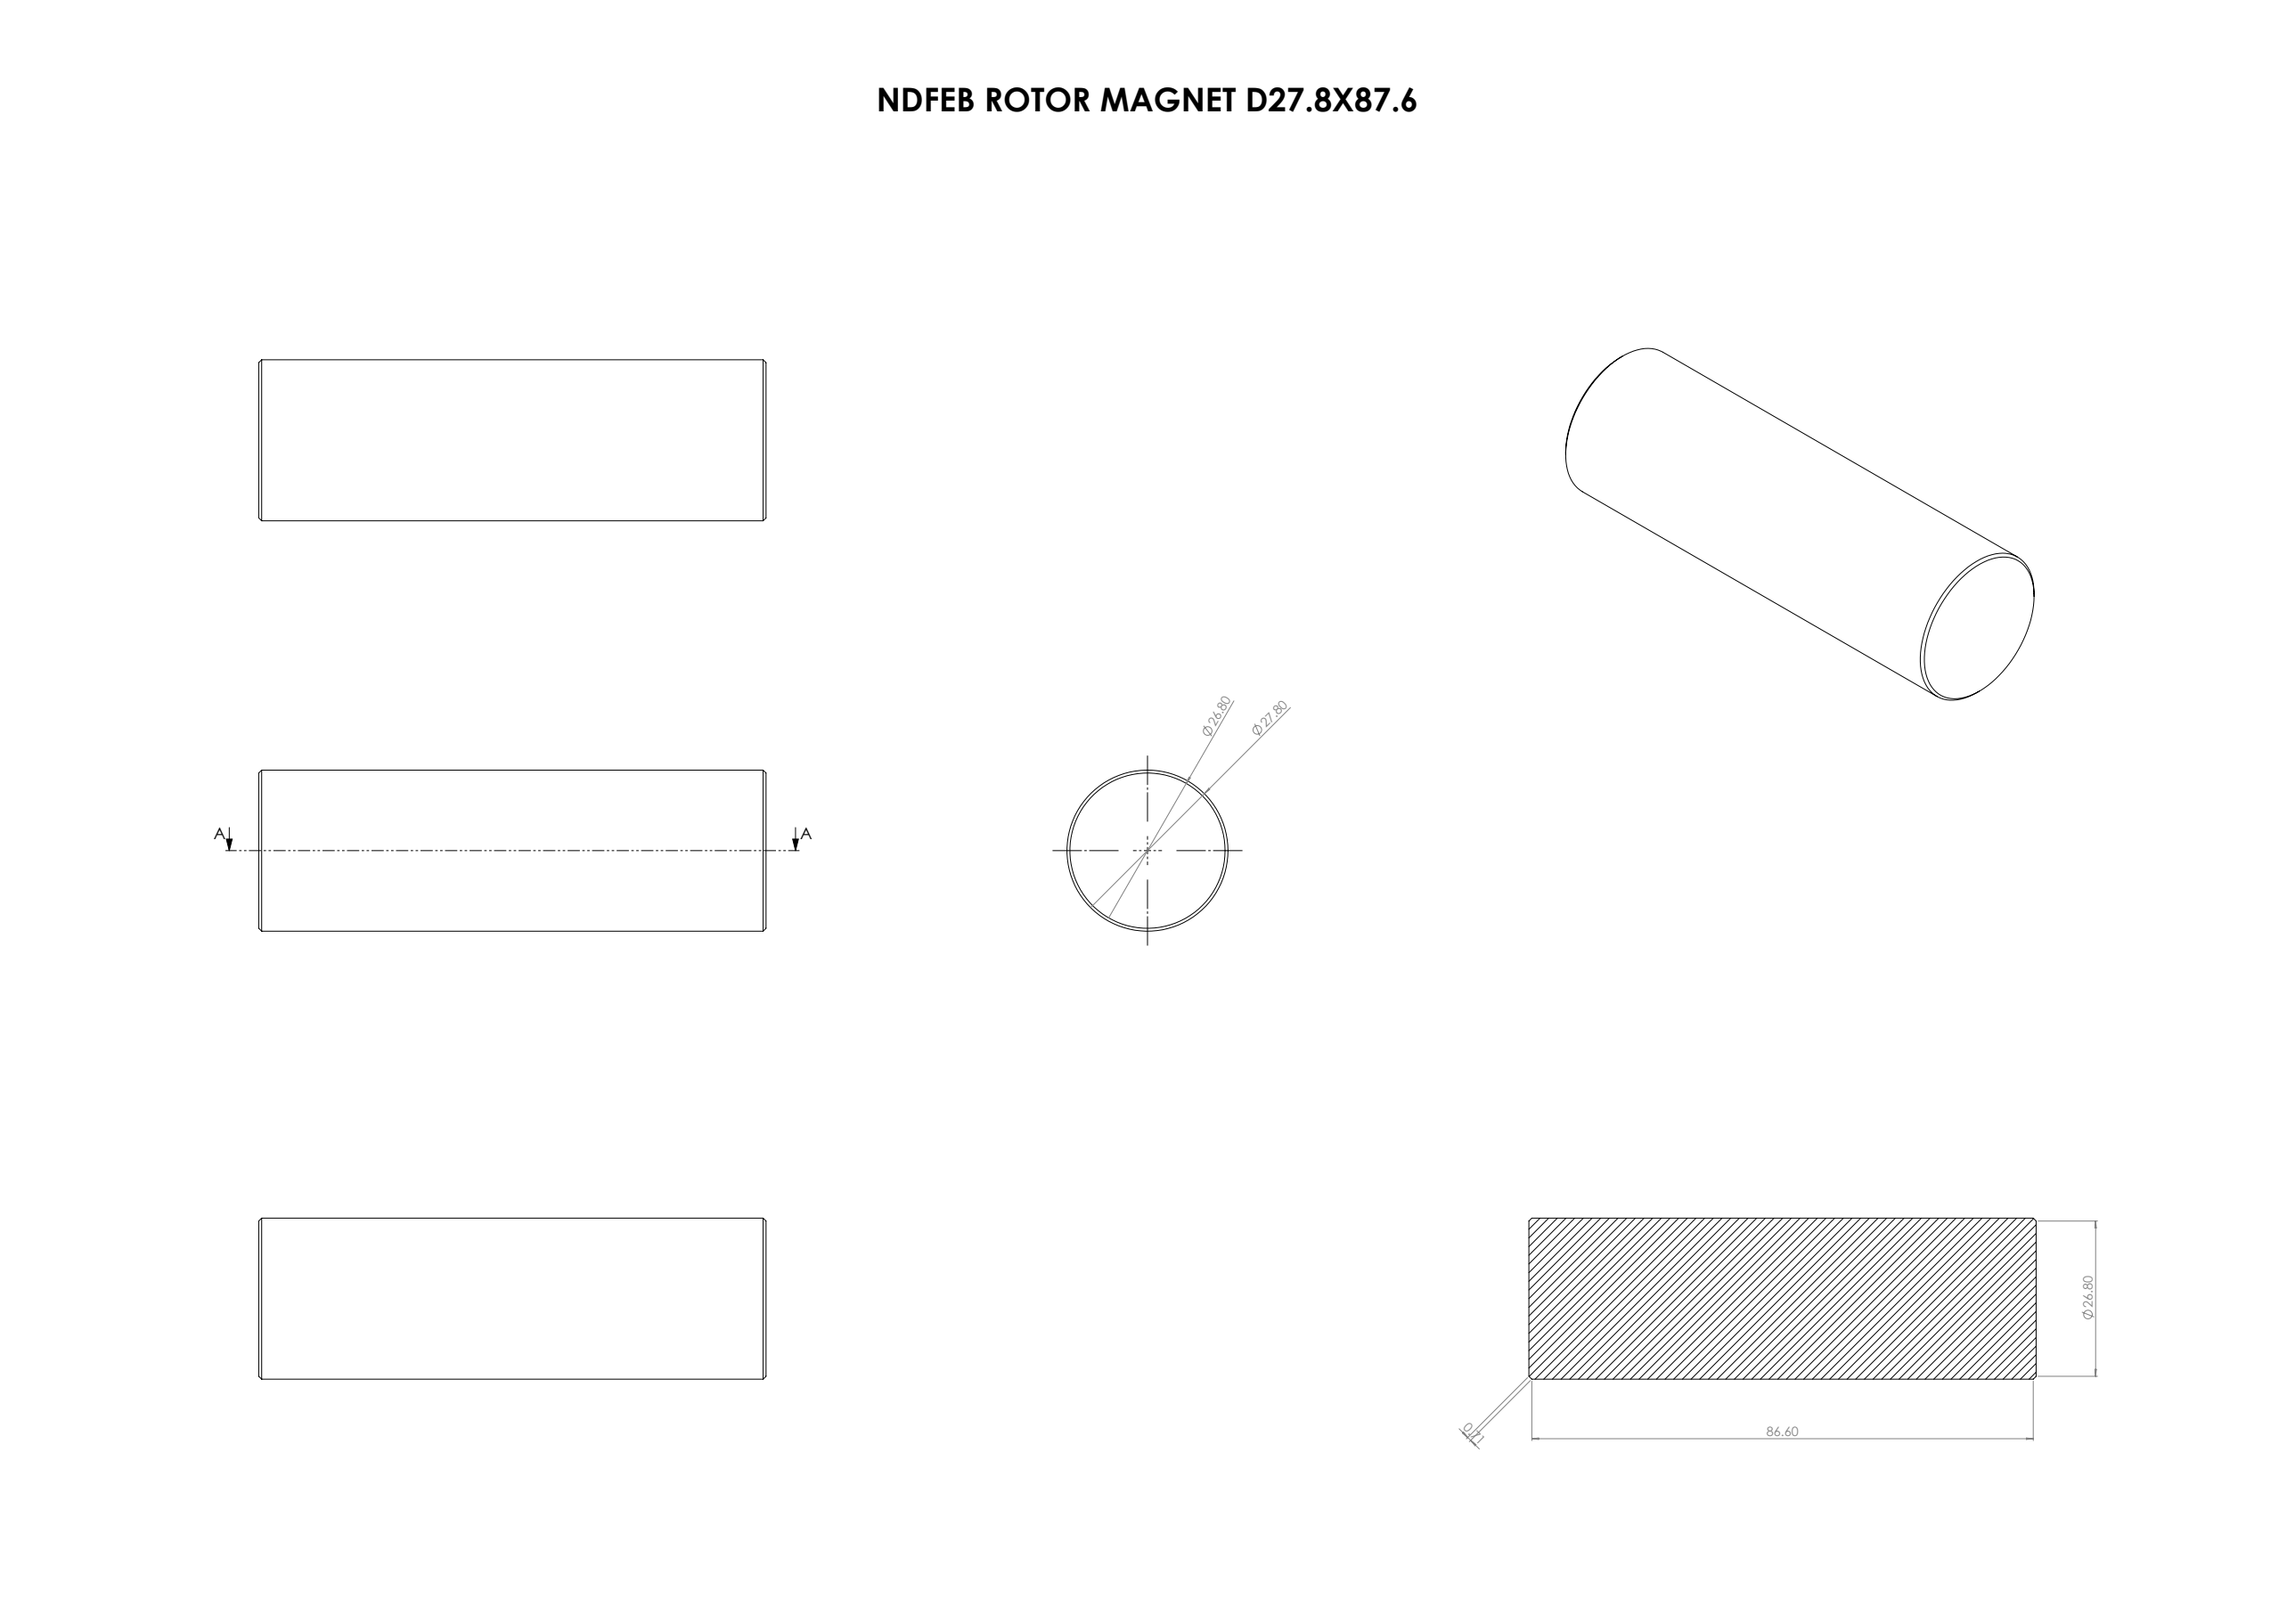
ISO-10303-21;
HEADER;
/* Generated by software containing ST-Developer
 * from STEP Tools, Inc. (www.steptools.com) 
 */

FILE_DESCRIPTION(
/* description */ (''),
/* implementation_level */ '2;1');

FILE_NAME(
/* name */ '03_NdFeB_Rotor_Magnet_D27.8x87.6.step',
/* time_stamp */ '2026-10-21T01:59:45-07:00',
/* author */ (''),
/* organization */ (''),
/* preprocessor_version */ 'ST-DEVELOPER v20.2',
/* originating_system */ 'Autodesk Translation Framework v15.15.0.0',
/* authorisation */ '');

FILE_SCHEMA (('AUTOMOTIVE_DESIGN { 1 0 10303 214 3 1 1 }'));
ENDSEC;

DATA;
#10=MECHANICAL_DESIGN_GEOMETRIC_PRESENTATION_REPRESENTATION('',(#473),#18281);
#412=CONICAL_SURFACE('',#9667,13.65,0.785398163397449);
#413=CONICAL_SURFACE('',#9671,13.65,0.785398163397442);
#442=SHAPE_REPRESENTATION_RELATIONSHIP('SRR','None',#18344,#455);
#455=ADVANCED_BREP_SHAPE_REPRESENTATION('',(#486),#18273);
#473=STYLED_ITEM('',(#18460),#486);
#486=MANIFOLD_SOLID_BREP('Body1',#9090);
#525=CYLINDRICAL_SURFACE('',#9669,13.9);
#733=CIRCLE('',#9666,13.4);
#734=CIRCLE('',#9668,13.9);
#735=CIRCLE('',#9670,13.9);
#736=CIRCLE('',#9672,13.4);
#1182=FACE_OUTER_BOUND('',#1743,.T.);
#1183=FACE_OUTER_BOUND('',#1744,.T.);
#1184=FACE_OUTER_BOUND('',#1745,.T.);
#1185=FACE_OUTER_BOUND('',#1746,.T.);
#1186=FACE_OUTER_BOUND('',#1747,.T.);
#1743=EDGE_LOOP('',(#7358));
#1744=EDGE_LOOP('',(#7359,#7360,#7361,#7362));
#1745=EDGE_LOOP('',(#7363,#7364,#7365,#7366));
#1746=EDGE_LOOP('',(#7367,#7368,#7369,#7370));
#1747=EDGE_LOOP('',(#7371));
#2550=LINE('',#14444,#3395);
#2551=LINE('',#14448,#3396);
#2552=LINE('',#14452,#3397);
#3395=VECTOR('',#11438,13.65);
#3396=VECTOR('',#11443,13.9);
#3397=VECTOR('',#11448,13.65);
#4136=VERTEX_POINT('',#14439);
#4137=VERTEX_POINT('',#14442);
#4138=VERTEX_POINT('',#14446);
#4139=VERTEX_POINT('',#14450);
#5251=EDGE_CURVE('',#4136,#4136,#733,.T.);
#5252=EDGE_CURVE('',#4137,#4137,#734,.T.);
#5253=EDGE_CURVE('',#4137,#4136,#2550,.T.);
#5254=EDGE_CURVE('',#4138,#4138,#735,.T.);
#5255=EDGE_CURVE('',#4138,#4137,#2551,.T.);
#5256=EDGE_CURVE('',#4139,#4139,#736,.T.);
#5257=EDGE_CURVE('',#4139,#4138,#2552,.T.);
#7358=ORIENTED_EDGE('',*,*,#5251,.F.);
#7359=ORIENTED_EDGE('',*,*,#5252,.F.);
#7360=ORIENTED_EDGE('',*,*,#5253,.T.);
#7361=ORIENTED_EDGE('',*,*,#5251,.T.);
#7362=ORIENTED_EDGE('',*,*,#5253,.F.);
#7363=ORIENTED_EDGE('',*,*,#5254,.F.);
#7364=ORIENTED_EDGE('',*,*,#5255,.T.);
#7365=ORIENTED_EDGE('',*,*,#5252,.T.);
#7366=ORIENTED_EDGE('',*,*,#5255,.F.);
#7367=ORIENTED_EDGE('',*,*,#5256,.F.);
#7368=ORIENTED_EDGE('',*,*,#5257,.T.);
#7369=ORIENTED_EDGE('',*,*,#5254,.T.);
#7370=ORIENTED_EDGE('',*,*,#5257,.F.);
#7371=ORIENTED_EDGE('',*,*,#5256,.T.);
#8465=PLANE('',#9665);
#8466=PLANE('',#9673);
#8903=ADVANCED_FACE('',(#1182),#8465,.T.);
#8904=ADVANCED_FACE('',(#1183),#412,.T.);
#8905=ADVANCED_FACE('',(#1184),#525,.T.);
#8906=ADVANCED_FACE('',(#1185),#413,.T.);
#8907=ADVANCED_FACE('',(#1186),#8466,.T.);
#9090=CLOSED_SHELL('',(#8903,#8904,#8905,#8906,#8907));
#9664=AXIS2_PLACEMENT_3D('',#14437,#11428,#11429);
#9665=AXIS2_PLACEMENT_3D('',#14438,#11430,#11431);
#9666=AXIS2_PLACEMENT_3D('',#14440,#11432,#11433);
#9667=AXIS2_PLACEMENT_3D('',#14441,#11434,#11435);
#9668=AXIS2_PLACEMENT_3D('',#14443,#11436,#11437);
#9669=AXIS2_PLACEMENT_3D('',#14445,#11439,#11440);
#9670=AXIS2_PLACEMENT_3D('',#14447,#11441,#11442);
#9671=AXIS2_PLACEMENT_3D('',#14449,#11444,#11445);
#9672=AXIS2_PLACEMENT_3D('',#14451,#11446,#11447);
#9673=AXIS2_PLACEMENT_3D('',#14453,#11449,#11450);
#11428=DIRECTION('axis',(0.,0.,1.));
#11429=DIRECTION('refdir',(1.,0.,0.));
#11430=DIRECTION('center_axis',(-1.,0.,0.));
#11431=DIRECTION('ref_axis',(0.,0.,1.));
#11432=DIRECTION('center_axis',(1.,0.,0.));
#11433=DIRECTION('ref_axis',(0.,0.,-1.));
#11434=DIRECTION('center_axis',(1.,0.,0.));
#11435=DIRECTION('ref_axis',(0.,1.,0.));
#11436=DIRECTION('center_axis',(1.,0.,0.));
#11437=DIRECTION('ref_axis',(0.,0.,-1.));
#11438=DIRECTION('',(-0.707106781186547,0.707106781186548,8.65956056235494E-17));
#11439=DIRECTION('center_axis',(1.,0.,0.));
#11440=DIRECTION('ref_axis',(0.,1.,0.));
#11441=DIRECTION('center_axis',(1.,0.,0.));
#11442=DIRECTION('ref_axis',(0.,0.,-1.));
#11443=DIRECTION('',(-1.,0.,0.));
#11444=DIRECTION('center_axis',(-1.,0.,0.));
#11445=DIRECTION('ref_axis',(0.,1.,0.));
#11446=DIRECTION('center_axis',(1.,0.,0.));
#11447=DIRECTION('ref_axis',(0.,0.,-1.));
#11448=DIRECTION('',(-0.707106781186552,-0.707106781186543,-8.65956056235488E-17));
#11449=DIRECTION('center_axis',(1.,0.,0.));
#11450=DIRECTION('ref_axis',(0.,0.,-1.));
#14437=CARTESIAN_POINT('',(0.,0.,0.));
#14438=CARTESIAN_POINT('Origin',(0.,13.4,0.));
#14439=CARTESIAN_POINT('',(9.0205620750794E-16,-13.4,-1.64102671085745E-15));
#14440=CARTESIAN_POINT('Origin',(0.,0.,0.));
#14441=CARTESIAN_POINT('Origin',(0.250000000000004,0.,0.));
#14442=CARTESIAN_POINT('',(0.500000000000005,-13.9,-1.70225905081482E-15));
#14443=CARTESIAN_POINT('Origin',(0.500000000000007,0.,0.));
#14444=CARTESIAN_POINT('',(0.250000000000004,-13.65,-1.67164288083614E-15));
#14445=CARTESIAN_POINT('Origin',(43.8,0.,0.));
#14446=CARTESIAN_POINT('',(87.1,-13.9,-1.70225905081482E-15));
#14447=CARTESIAN_POINT('Origin',(87.1,0.,0.));
#14448=CARTESIAN_POINT('',(43.8,-13.9,-1.70225905081482E-15));
#14449=CARTESIAN_POINT('Origin',(87.35,0.,0.));
#14450=CARTESIAN_POINT('',(87.6,-13.4,-1.64102671085745E-15));
#14451=CARTESIAN_POINT('Origin',(87.6,0.,0.));
#14452=CARTESIAN_POINT('',(87.35,-13.65,-1.67164288083614E-15));
#14453=CARTESIAN_POINT('Origin',(87.6,0.,0.));
#18258=UNCERTAINTY_MEASURE_WITH_UNIT(LENGTH_MEASURE(0.01),#18282,
'DISTANCE_ACCURACY_VALUE',
'Maximum model space distance between geometric entities at asserted c
onnectivities');
#18266=UNCERTAINTY_MEASURE_WITH_UNIT(LENGTH_MEASURE(0.01),#18282,
'DISTANCE_ACCURACY_VALUE',
'Maximum model space distance between geometric entities at asserted c
onnectivities');
#18273=(
GEOMETRIC_REPRESENTATION_CONTEXT(3)
GLOBAL_UNCERTAINTY_ASSIGNED_CONTEXT((#18258))
GLOBAL_UNIT_ASSIGNED_CONTEXT((#18282,#18284,#18285))
REPRESENTATION_CONTEXT('','3D')
);
#18281=(
GEOMETRIC_REPRESENTATION_CONTEXT(3)
GLOBAL_UNCERTAINTY_ASSIGNED_CONTEXT((#18266))
GLOBAL_UNIT_ASSIGNED_CONTEXT((#18282,#18284,#18285))
REPRESENTATION_CONTEXT('','3D')
);
#18282=(
LENGTH_UNIT()
NAMED_UNIT(*)
SI_UNIT(.MILLI.,.METRE.)
);
#18284=(
NAMED_UNIT(*)
PLANE_ANGLE_UNIT()
SI_UNIT($,.RADIAN.)
);
#18285=(
NAMED_UNIT(*)
SI_UNIT($,.STERADIAN.)
SOLID_ANGLE_UNIT()
);
#18292=SHAPE_DEFINITION_REPRESENTATION(#18306,#18344);
#18306=PRODUCT_DEFINITION_SHAPE('',$,#18359);
#18344=SHAPE_REPRESENTATION('',(#9664),#18273);
#18352=PRODUCT_DEFINITION_CONTEXT('part definition',#18396,'design');
#18359=PRODUCT_DEFINITION('2026-10-20-13-03-18-366',
'03_NdFeB_Rotor_Magnet_D27.8x87.6',#18373,#18352);
#18373=PRODUCT_DEFINITION_FORMATION('',$,#18404);
#18396=APPLICATION_CONTEXT(
'Core Data for Automotive Mechanical Design Process');
#18397=PRODUCT_CONTEXT('part definition',#18396,'mechanical');
#18404=PRODUCT('2026-10-20-13-03-18-366',
'03_NdFeB_Rotor_Magnet_D27.8x87.6',$,(#18397));
#18454=COLOUR_RGB('Light Blue',0.38,0.62,0.78);
#18455=FILL_AREA_STYLE_COLOUR('',#18454);
#18456=FILL_AREA_STYLE('',(#18455));
#18457=SURFACE_STYLE_FILL_AREA(#18456);
#18458=SURFACE_SIDE_STYLE('',(#18457));
#18459=SURFACE_STYLE_USAGE(.BOTH.,#18458);
#18460=PRESENTATION_STYLE_ASSIGNMENT((#18459));
ENDSEC;
END-ISO-10303-21;
